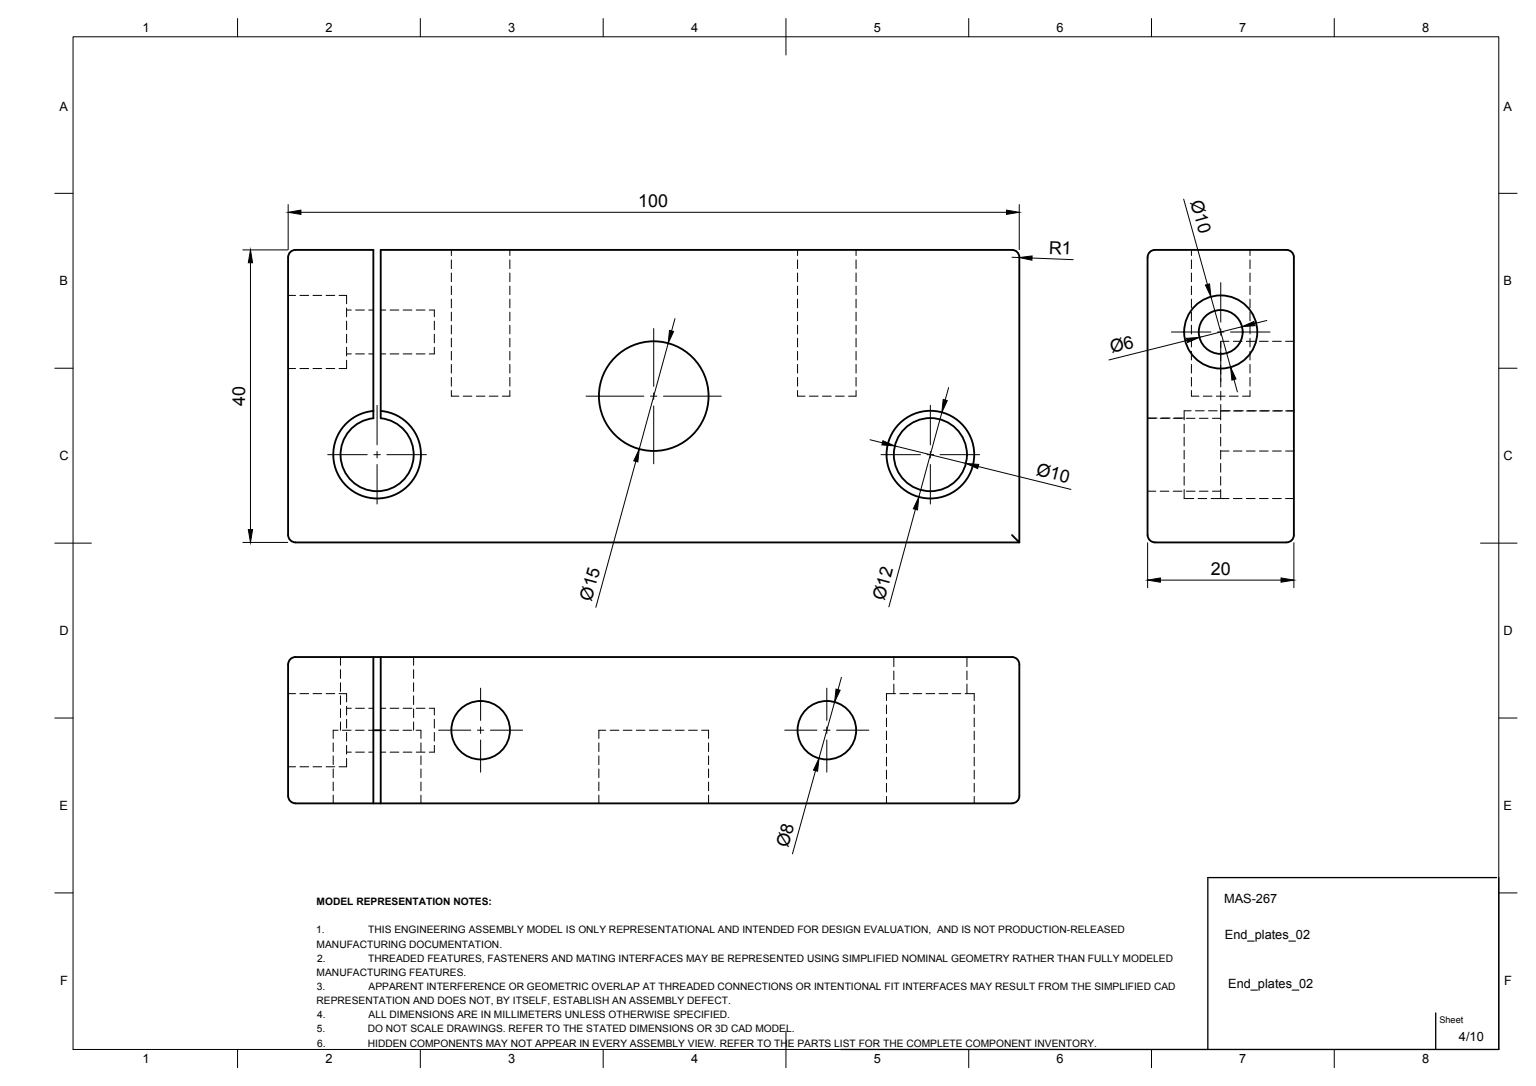
ISO-10303-21;
HEADER;
/* Generated by software containing ST-Developer
 * from STEP Tools, Inc. (www.steptools.com) 
 */

FILE_DESCRIPTION(
/* description */ (''),
/* implementation_level */ '2;1');

FILE_NAME(
/* name */ 'End_plates_02.step',
/* time_stamp */ '2026-10-12T15:29:24-07:00',
/* author */ (''),
/* organization */ (''),
/* preprocessor_version */ 'ST-DEVELOPER v20.2',
/* originating_system */ 'Autodesk Translation Framework v15.15.0.0',
/* authorisation */ '');

FILE_SCHEMA (('AUTOMOTIVE_DESIGN { 1 0 10303 214 3 1 1 }'));
ENDSEC;

DATA;
#10=MECHANICAL_DESIGN_GEOMETRIC_PRESENTATION_REPRESENTATION('',(#163),#9496);
#145=SHAPE_REPRESENTATION_RELATIONSHIP('SRR','None',#9539,#154);
#154=ADVANCED_BREP_SHAPE_REPRESENTATION('',(#220),#9487);
#163=STYLED_ITEM('',(#9593),#220);
#220=MANIFOLD_SOLID_BREP('Body1',#4965);
#277=ELLIPSE('',#5185,1.4142135623731,1.);
#278=ELLIPSE('',#5196,1.4142135623731,1.);
#279=SPHERICAL_SURFACE('',#5169,0.999999999999996);
#280=SPHERICAL_SURFACE('',#5173,0.999999999999996);
#281=SPHERICAL_SURFACE('',#5177,0.999999999999996);
#282=SPHERICAL_SURFACE('',#5181,0.999999999999996);
#283=SPHERICAL_SURFACE('',#5186,0.999999999999996);
#284=SPHERICAL_SURFACE('',#5192,0.999999999999996);
#333=FACE_BOUND('',#956,.T.);
#334=FACE_BOUND('',#963,.T.);
#335=FACE_BOUND('',#970,.T.);
#336=FACE_BOUND('',#972,.T.);
#337=FACE_BOUND('',#975,.T.);
#338=FACE_BOUND('',#978,.T.);
#339=FACE_BOUND('',#979,.T.);
#340=FACE_BOUND('',#1000,.T.);
#341=FACE_BOUND('',#1001,.T.);
#342=FACE_BOUND('',#1003,.T.);
#482=PLANE('',#5127);
#483=PLANE('',#5132);
#484=PLANE('',#5136);
#485=PLANE('',#5140);
#486=PLANE('',#5147);
#487=PLANE('',#5153);
#488=PLANE('',#5154);
#489=PLANE('',#5157);
#490=PLANE('',#5159);
#491=PLANE('',#5164);
#492=PLANE('',#5202);
#493=PLANE('',#5203);
#494=PLANE('',#5206);
#495=PLANE('',#5207);
#496=PLANE('',#5209);
#497=PLANE('',#5212);
#622=FACE_OUTER_BOUND('',#954,.T.);
#623=FACE_OUTER_BOUND('',#955,.T.);
#624=FACE_OUTER_BOUND('',#957,.T.);
#625=FACE_OUTER_BOUND('',#958,.T.);
#626=FACE_OUTER_BOUND('',#959,.T.);
#627=FACE_OUTER_BOUND('',#960,.T.);
#628=FACE_OUTER_BOUND('',#961,.T.);
#629=FACE_OUTER_BOUND('',#962,.T.);
#630=FACE_OUTER_BOUND('',#964,.T.);
#631=FACE_OUTER_BOUND('',#965,.T.);
#632=FACE_OUTER_BOUND('',#966,.T.);
#633=FACE_OUTER_BOUND('',#967,.T.);
#634=FACE_OUTER_BOUND('',#968,.T.);
#635=FACE_OUTER_BOUND('',#969,.T.);
#636=FACE_OUTER_BOUND('',#971,.T.);
#637=FACE_OUTER_BOUND('',#973,.T.);
#638=FACE_OUTER_BOUND('',#974,.T.);
#639=FACE_OUTER_BOUND('',#976,.T.);
#640=FACE_OUTER_BOUND('',#977,.T.);
#641=FACE_OUTER_BOUND('',#980,.T.);
#642=FACE_OUTER_BOUND('',#981,.T.);
#643=FACE_OUTER_BOUND('',#982,.T.);
#644=FACE_OUTER_BOUND('',#983,.T.);
#645=FACE_OUTER_BOUND('',#984,.T.);
#646=FACE_OUTER_BOUND('',#985,.T.);
#647=FACE_OUTER_BOUND('',#986,.T.);
#648=FACE_OUTER_BOUND('',#987,.T.);
#649=FACE_OUTER_BOUND('',#988,.T.);
#650=FACE_OUTER_BOUND('',#989,.T.);
#651=FACE_OUTER_BOUND('',#990,.T.);
#652=FACE_OUTER_BOUND('',#991,.T.);
#653=FACE_OUTER_BOUND('',#992,.T.);
#654=FACE_OUTER_BOUND('',#993,.T.);
#655=FACE_OUTER_BOUND('',#994,.T.);
#656=FACE_OUTER_BOUND('',#995,.T.);
#657=FACE_OUTER_BOUND('',#996,.T.);
#658=FACE_OUTER_BOUND('',#997,.T.);
#659=FACE_OUTER_BOUND('',#998,.T.);
#660=FACE_OUTER_BOUND('',#999,.T.);
#661=FACE_OUTER_BOUND('',#1002,.T.);
#662=FACE_OUTER_BOUND('',#1004,.T.);
#663=FACE_OUTER_BOUND('',#1005,.T.);
#664=FACE_OUTER_BOUND('',#1006,.T.);
#665=FACE_OUTER_BOUND('',#1007,.T.);
#666=FACE_OUTER_BOUND('',#1008,.T.);
#954=EDGE_LOOP('',(#3325,#3326,#3327,#3328));
#955=EDGE_LOOP('',(#3329));
#956=EDGE_LOOP('',(#3330));
#957=EDGE_LOOP('',(#3331,#3332,#3333,#3334));
#958=EDGE_LOOP('',(#3335));
#959=EDGE_LOOP('',(#3336,#3337,#3338,#3339));
#960=EDGE_LOOP('',(#3340));
#961=EDGE_LOOP('',(#3341,#3342,#3343,#3344));
#962=EDGE_LOOP('',(#3345));
#963=EDGE_LOOP('',(#3346));
#964=EDGE_LOOP('',(#3347,#3348,#3349,#3350));
#965=EDGE_LOOP('',(#3351,#3352,#3353,#3354));
#966=EDGE_LOOP('',(#3355));
#967=EDGE_LOOP('',(#3356,#3357,#3358,#3359));
#968=EDGE_LOOP('',(#3360,#3361,#3362,#3363));
#969=EDGE_LOOP('',(#3364,#3365,#3366,#3367,#3368,#3369,#3370,#3371));
#970=EDGE_LOOP('',(#3372));
#971=EDGE_LOOP('',(#3373,#3374,#3375,#3376,#3377,#3378,#3379,#3380));
#972=EDGE_LOOP('',(#3381));
#973=EDGE_LOOP('',(#3382,#3383,#3384,#3385));
#974=EDGE_LOOP('',(#3386,#3387,#3388,#3389,#3390,#3391,#3392,#3393));
#975=EDGE_LOOP('',(#3394));
#976=EDGE_LOOP('',(#3395,#3396,#3397,#3398));
#977=EDGE_LOOP('',(#3399,#3400,#3401,#3402));
#978=EDGE_LOOP('',(#3403));
#979=EDGE_LOOP('',(#3404));
#980=EDGE_LOOP('',(#3405,#3406,#3407,#3408));
#981=EDGE_LOOP('',(#3409,#3410,#3411,#3412));
#982=EDGE_LOOP('',(#3413,#3414,#3415));
#983=EDGE_LOOP('',(#3416,#3417,#3418));
#984=EDGE_LOOP('',(#3419,#3420,#3421,#3422));
#985=EDGE_LOOP('',(#3423,#3424,#3425));
#986=EDGE_LOOP('',(#3426,#3427,#3428));
#987=EDGE_LOOP('',(#3429,#3430,#3431,#3432));
#988=EDGE_LOOP('',(#3433,#3434,#3435));
#989=EDGE_LOOP('',(#3436,#3437,#3438,#3439));
#990=EDGE_LOOP('',(#3440,#3441,#3442,#3443));
#991=EDGE_LOOP('',(#3444,#3445,#3446));
#992=EDGE_LOOP('',(#3447,#3448,#3449,#3450));
#993=EDGE_LOOP('',(#3451,#3452,#3453,#3454));
#994=EDGE_LOOP('',(#3455,#3456,#3457,#3458));
#995=EDGE_LOOP('',(#3459,#3460,#3461,#3462));
#996=EDGE_LOOP('',(#3463,#3464,#3465,#3466));
#997=EDGE_LOOP('',(#3467,#3468,#3469,#3470));
#998=EDGE_LOOP('',(#3471,#3472,#3473,#3474));
#999=EDGE_LOOP('',(#3475,#3476,#3477,#3478,#3479,#3480,#3481,#3482));
#1000=EDGE_LOOP('',(#3483));
#1001=EDGE_LOOP('',(#3484));
#1002=EDGE_LOOP('',(#3485,#3486,#3487,#3488));
#1003=EDGE_LOOP('',(#3489));
#1004=EDGE_LOOP('',(#3490,#3491,#3492,#3493));
#1005=EDGE_LOOP('',(#3494,#3495,#3496,#3497));
#1006=EDGE_LOOP('',(#3498));
#1007=EDGE_LOOP('',(#3499,#3500,#3501,#3502));
#1008=EDGE_LOOP('',(#3503,#3504,#3505,#3506));
#1435=LINE('',#7477,#1672);
#1436=LINE('',#7486,#1673);
#1437=LINE('',#7493,#1674);
#1438=LINE('',#7500,#1675);
#1439=LINE('',#7507,#1676);
#1440=LINE('',#7513,#1677);
#1441=LINE('',#7518,#1678);
#1442=LINE('',#7523,#1679);
#1443=LINE('',#7527,#1680);
#1444=LINE('',#7531,#1681);
#1445=LINE('',#7533,#1682);
#1446=LINE('',#7535,#1683);
#1447=LINE('',#7537,#1684);
#1448=LINE('',#7539,#1685);
#1449=LINE('',#7541,#1686);
#1450=LINE('',#7542,#1687);
#1451=LINE('',#7545,#1688);
#1452=LINE('',#7547,#1689);
#1453=LINE('',#7549,#1690);
#1454=LINE('',#7553,#1691);
#1455=LINE('',#7557,#1692);
#1456=LINE('',#7563,#1693);
#1457=LINE('',#7567,#1694);
#1458=LINE('',#7568,#1695);
#1459=LINE('',#7571,#1696);
#1460=LINE('',#7575,#1697);
#1461=LINE('',#7576,#1698);
#1462=LINE('',#7579,#1699);
#1463=LINE('',#7583,#1700);
#1464=LINE('',#7586,#1701);
#1465=LINE('',#7599,#1702);
#1466=LINE('',#7600,#1703);
#1467=LINE('',#7613,#1704);
#1468=LINE('',#7615,#1705);
#1469=LINE('',#7624,#1706);
#1470=LINE('',#7626,#1707);
#1471=LINE('',#7627,#1708);
#1472=LINE('',#7634,#1709);
#1473=LINE('',#7637,#1710);
#1474=LINE('',#7639,#1711);
#1475=LINE('',#7641,#1712);
#1476=LINE('',#7643,#1713);
#1477=LINE('',#7644,#1714);
#1478=LINE('',#7646,#1715);
#1479=LINE('',#7647,#1716);
#1480=LINE('',#7649,#1717);
#1481=LINE('',#7661,#1718);
#1672=VECTOR('',#5834,6.00000000000001);
#1673=VECTOR('',#5845,4.);
#1674=VECTOR('',#5854,4.);
#1675=VECTOR('',#5863,5.);
#1676=VECTOR('',#5872,3.00000000000001);
#1677=VECTOR('',#5879,3.00000000000001);
#1678=VECTOR('',#5886,4.99999999999977);
#1679=VECTOR('',#5891,10.);
#1680=VECTOR('',#5894,10.);
#1681=VECTOR('',#5899,10.);
#1682=VECTOR('',#5900,10.);
#1683=VECTOR('',#5901,10.);
#1684=VECTOR('',#5902,10.);
#1685=VECTOR('',#5903,10.);
#1686=VECTOR('',#5904,10.);
#1687=VECTOR('',#5905,10.);
#1688=VECTOR('',#5908,10.);
#1689=VECTOR('',#5909,10.);
#1690=VECTOR('',#5910,10.);
#1691=VECTOR('',#5913,10.);
#1692=VECTOR('',#5918,10.);
#1693=VECTOR('',#5925,10.);
#1694=VECTOR('',#5928,10.);
#1695=VECTOR('',#5929,10.);
#1696=VECTOR('',#5932,10.);
#1697=VECTOR('',#5937,10.);
#1698=VECTOR('',#5938,10.);
#1699=VECTOR('',#5941,10.);
#1700=VECTOR('',#5946,10.);
#1701=VECTOR('',#5949,10.);
#1702=VECTOR('',#5966,10.);
#1703=VECTOR('',#5967,10.);
#1704=VECTOR('',#5984,10.);
#1705=VECTOR('',#5985,10.);
#1706=VECTOR('',#5998,10.);
#1707=VECTOR('',#6001,10.);
#1708=VECTOR('',#6002,10.);
#1709=VECTOR('',#6011,10.);
#1710=VECTOR('',#6016,10.);
#1711=VECTOR('',#6019,10.);
#1712=VECTOR('',#6022,10.);
#1713=VECTOR('',#6025,10.);
#1714=VECTOR('',#6026,10.);
#1715=VECTOR('',#6029,10.);
#1716=VECTOR('',#6030,10.);
#1717=VECTOR('',#6033,10.);
#1718=VECTOR('',#6052,7.50000000000001);
#1909=CIRCLE('',#5125,6.00000000000001);
#1910=CIRCLE('',#5126,6.00000000000001);
#1911=CIRCLE('',#5128,4.99999999999977);
#1912=CIRCLE('',#5130,4.);
#1913=CIRCLE('',#5131,4.);
#1914=CIRCLE('',#5134,4.);
#1915=CIRCLE('',#5135,4.);
#1916=CIRCLE('',#5138,5.);
#1917=CIRCLE('',#5139,5.);
#1918=CIRCLE('',#5141,3.00000000000001);
#1919=CIRCLE('',#5143,3.00000000000001);
#1920=CIRCLE('',#5145,3.00000000000001);
#1921=CIRCLE('',#5146,3.00000000000001);
#1922=CIRCLE('',#5149,4.99999999999977);
#1923=CIRCLE('',#5151,4.99999999999977);
#1924=CIRCLE('',#5152,4.99999999999977);
#1925=CIRCLE('',#5155,1.);
#1926=CIRCLE('',#5156,1.);
#1927=CIRCLE('',#5158,6.00000000000001);
#1928=CIRCLE('',#5160,1.);
#1929=CIRCLE('',#5161,1.);
#1930=CIRCLE('',#5163,1.);
#1931=CIRCLE('',#5166,0.999999999999996);
#1932=CIRCLE('',#5168,1.);
#1933=CIRCLE('',#5170,0.999999999999996);
#1934=CIRCLE('',#5171,0.999999999999996);
#1935=CIRCLE('',#5172,1.);
#1936=CIRCLE('',#5174,0.999999999999996);
#1937=CIRCLE('',#5175,0.999999999999996);
#1938=CIRCLE('',#5178,0.999999999999996);
#1939=CIRCLE('',#5179,0.999999999999996);
#1940=CIRCLE('',#5180,1.);
#1941=CIRCLE('',#5182,0.999999999999996);
#1942=CIRCLE('',#5183,1.);
#1943=CIRCLE('',#5187,0.999999999999996);
#1944=CIRCLE('',#5188,0.999999999999996);
#1945=CIRCLE('',#5189,1.);
#1946=CIRCLE('',#5193,0.999999999999996);
#1947=CIRCLE('',#5194,0.999999999999996);
#1948=CIRCLE('',#5204,6.00000000000001);
#1949=CIRCLE('',#5205,7.50000000000001);
#1950=CIRCLE('',#5210,7.50000000000001);
#2264=VERTEX_POINT('',#7474);
#2265=VERTEX_POINT('',#7476);
#2266=VERTEX_POINT('',#7480);
#2267=VERTEX_POINT('',#7483);
#2268=VERTEX_POINT('',#7485);
#2269=VERTEX_POINT('',#7490);
#2270=VERTEX_POINT('',#7492);
#2271=VERTEX_POINT('',#7497);
#2272=VERTEX_POINT('',#7499);
#2273=VERTEX_POINT('',#7503);
#2274=VERTEX_POINT('',#7506);
#2275=VERTEX_POINT('',#7510);
#2276=VERTEX_POINT('',#7512);
#2277=VERTEX_POINT('',#7517);
#2278=VERTEX_POINT('',#7521);
#2279=VERTEX_POINT('',#7522);
#2280=VERTEX_POINT('',#7524);
#2281=VERTEX_POINT('',#7526);
#2282=VERTEX_POINT('',#7530);
#2283=VERTEX_POINT('',#7532);
#2284=VERTEX_POINT('',#7534);
#2285=VERTEX_POINT('',#7536);
#2286=VERTEX_POINT('',#7538);
#2287=VERTEX_POINT('',#7540);
#2288=VERTEX_POINT('',#7544);
#2289=VERTEX_POINT('',#7546);
#2290=VERTEX_POINT('',#7548);
#2291=VERTEX_POINT('',#7550);
#2292=VERTEX_POINT('',#7552);
#2293=VERTEX_POINT('',#7556);
#2294=VERTEX_POINT('',#7560);
#2295=VERTEX_POINT('',#7562);
#2296=VERTEX_POINT('',#7564);
#2297=VERTEX_POINT('',#7566);
#2298=VERTEX_POINT('',#7570);
#2299=VERTEX_POINT('',#7574);
#2300=VERTEX_POINT('',#7578);
#2301=VERTEX_POINT('',#7582);
#2302=VERTEX_POINT('',#7584);
#2303=VERTEX_POINT('',#7588);
#2304=VERTEX_POINT('',#7589);
#2305=VERTEX_POINT('',#7591);
#2306=VERTEX_POINT('',#7595);
#2307=VERTEX_POINT('',#7602);
#2308=VERTEX_POINT('',#7603);
#2309=VERTEX_POINT('',#7608);
#2310=VERTEX_POINT('',#7612);
#2311=VERTEX_POINT('',#7614);
#2312=VERTEX_POINT('',#7618);
#2313=VERTEX_POINT('',#7620);
#2314=VERTEX_POINT('',#7629);
#2315=VERTEX_POINT('',#7633);
#2316=VERTEX_POINT('',#7652);
#2317=VERTEX_POINT('',#7658);
#2715=EDGE_CURVE('',#2264,#2264,#1909,.T.);
#2716=EDGE_CURVE('',#2264,#2265,#1435,.T.);
#2717=EDGE_CURVE('',#2265,#2265,#1910,.T.);
#2718=EDGE_CURVE('',#2266,#2266,#1911,.T.);
#2719=EDGE_CURVE('',#2267,#2267,#1912,.T.);
#2720=EDGE_CURVE('',#2267,#2268,#1436,.T.);
#2721=EDGE_CURVE('',#2268,#2268,#1913,.T.);
#2722=EDGE_CURVE('',#2269,#2269,#1914,.T.);
#2723=EDGE_CURVE('',#2269,#2270,#1437,.T.);
#2724=EDGE_CURVE('',#2270,#2270,#1915,.T.);
#2725=EDGE_CURVE('',#2271,#2271,#1916,.T.);
#2726=EDGE_CURVE('',#2271,#2272,#1438,.T.);
#2727=EDGE_CURVE('',#2272,#2272,#1917,.T.);
#2728=EDGE_CURVE('',#2273,#2273,#1918,.T.);
#2729=EDGE_CURVE('',#2273,#2274,#1439,.T.);
#2730=EDGE_CURVE('',#2274,#2274,#1919,.T.);
#2731=EDGE_CURVE('',#2275,#2275,#1920,.T.);
#2732=EDGE_CURVE('',#2275,#2276,#1440,.T.);
#2733=EDGE_CURVE('',#2276,#2276,#1921,.T.);
#2734=EDGE_CURVE('',#2266,#2277,#1441,.T.);
#2735=EDGE_CURVE('',#2277,#2277,#1922,.T.);
#2736=EDGE_CURVE('',#2278,#2279,#1442,.T.);
#2737=EDGE_CURVE('',#2280,#2278,#1923,.T.);
#2738=EDGE_CURVE('',#2281,#2280,#1443,.T.);
#2739=EDGE_CURVE('',#2279,#2281,#1924,.T.);
#2740=EDGE_CURVE('',#2281,#2282,#1444,.T.);
#2741=EDGE_CURVE('',#2283,#2282,#1445,.T.);
#2742=EDGE_CURVE('',#2284,#2283,#1446,.T.);
#2743=EDGE_CURVE('',#2285,#2284,#1447,.T.);
#2744=EDGE_CURVE('',#2286,#2285,#1448,.T.);
#2745=EDGE_CURVE('',#2287,#2286,#1449,.T.);
#2746=EDGE_CURVE('',#2287,#2279,#1450,.T.);
#2747=EDGE_CURVE('',#2288,#2280,#1451,.T.);
#2748=EDGE_CURVE('',#2289,#2288,#1452,.T.);
#2749=EDGE_CURVE('',#2290,#2289,#1453,.T.);
#2750=EDGE_CURVE('',#2291,#2290,#1925,.T.);
#2751=EDGE_CURVE('',#2292,#2291,#1454,.T.);
#2752=EDGE_CURVE('',#2282,#2292,#1926,.T.);
#2753=EDGE_CURVE('',#2278,#2293,#1455,.T.);
#2754=EDGE_CURVE('',#2288,#2293,#1927,.T.);
#2755=EDGE_CURVE('',#2294,#2287,#1928,.T.);
#2756=EDGE_CURVE('',#2295,#2294,#1456,.T.);
#2757=EDGE_CURVE('',#2296,#2295,#1929,.T.);
#2758=EDGE_CURVE('',#2297,#2296,#1457,.T.);
#2759=EDGE_CURVE('',#2293,#2297,#1458,.T.);
#2760=EDGE_CURVE('',#2292,#2298,#1459,.T.);
#2761=EDGE_CURVE('',#2298,#2283,#1930,.F.);
#2762=EDGE_CURVE('',#2299,#2291,#1460,.T.);
#2763=EDGE_CURVE('',#2298,#2299,#1461,.T.);
#2764=EDGE_CURVE('',#2290,#2300,#1462,.T.);
#2765=EDGE_CURVE('',#2300,#2299,#1931,.F.);
#2766=EDGE_CURVE('',#2295,#2301,#1463,.T.);
#2767=EDGE_CURVE('',#2301,#2302,#1932,.F.);
#2768=EDGE_CURVE('',#2302,#2296,#1464,.T.);
#2769=EDGE_CURVE('',#2303,#2304,#1933,.F.);
#2770=EDGE_CURVE('',#2305,#2303,#1934,.F.);
#2771=EDGE_CURVE('',#2304,#2305,#1935,.F.);
#2772=EDGE_CURVE('',#2306,#2301,#1936,.F.);
#2773=EDGE_CURVE('',#2302,#2306,#1937,.F.);
#2774=EDGE_CURVE('',#2306,#2305,#1465,.T.);
#2775=EDGE_CURVE('',#2303,#2302,#1466,.T.);
#2776=EDGE_CURVE('',#2307,#2308,#1938,.F.);
#2777=EDGE_CURVE('',#2285,#2307,#1939,.F.);
#2778=EDGE_CURVE('',#2308,#2285,#1940,.F.);
#2779=EDGE_CURVE('',#2309,#2300,#1941,.F.);
#2780=EDGE_CURVE('',#2299,#2309,#1942,.F.);
#2781=EDGE_CURVE('',#2310,#2309,#1467,.T.);
#2782=EDGE_CURVE('',#2300,#2311,#1468,.T.);
#2783=EDGE_CURVE('',#2311,#2310,#277,.T.);
#2784=EDGE_CURVE('',#2286,#2312,#1943,.F.);
#2785=EDGE_CURVE('',#2313,#2286,#1944,.F.);
#2786=EDGE_CURVE('',#2312,#2313,#1945,.F.);
#2787=EDGE_CURVE('',#2307,#2313,#1469,.T.);
#2788=EDGE_CURVE('',#2301,#2312,#1470,.T.);
#2789=EDGE_CURVE('',#2313,#2306,#1471,.T.);
#2790=EDGE_CURVE('',#2314,#2298,#1946,.F.);
#2791=EDGE_CURVE('',#2283,#2314,#1947,.F.);
#2792=EDGE_CURVE('',#2314,#2315,#1472,.T.);
#2793=EDGE_CURVE('',#2315,#2284,#278,.T.);
#2794=EDGE_CURVE('',#2312,#2294,#1473,.T.);
#2795=EDGE_CURVE('',#2309,#2314,#1474,.T.);
#2796=EDGE_CURVE('',#2315,#2308,#1475,.T.);
#2797=EDGE_CURVE('',#2308,#2304,#1476,.T.);
#2798=EDGE_CURVE('',#2305,#2307,#1477,.T.);
#2799=EDGE_CURVE('',#2311,#2303,#1478,.T.);
#2800=EDGE_CURVE('',#2304,#2310,#1479,.T.);
#2801=EDGE_CURVE('',#2315,#2310,#1480,.T.);
#2802=EDGE_CURVE('',#2289,#2297,#1948,.T.);
#2803=EDGE_CURVE('',#2316,#2316,#1949,.T.);
#2804=EDGE_CURVE('',#2317,#2317,#1950,.T.);
#2805=EDGE_CURVE('',#2317,#2316,#1481,.T.);
#3325=ORIENTED_EDGE('',*,*,#2715,.F.);
#3326=ORIENTED_EDGE('',*,*,#2716,.T.);
#3327=ORIENTED_EDGE('',*,*,#2717,.T.);
#3328=ORIENTED_EDGE('',*,*,#2716,.F.);
#3329=ORIENTED_EDGE('',*,*,#2717,.F.);
#3330=ORIENTED_EDGE('',*,*,#2718,.F.);
#3331=ORIENTED_EDGE('',*,*,#2719,.F.);
#3332=ORIENTED_EDGE('',*,*,#2720,.T.);
#3333=ORIENTED_EDGE('',*,*,#2721,.T.);
#3334=ORIENTED_EDGE('',*,*,#2720,.F.);
#3335=ORIENTED_EDGE('',*,*,#2721,.F.);
#3336=ORIENTED_EDGE('',*,*,#2722,.F.);
#3337=ORIENTED_EDGE('',*,*,#2723,.T.);
#3338=ORIENTED_EDGE('',*,*,#2724,.T.);
#3339=ORIENTED_EDGE('',*,*,#2723,.F.);
#3340=ORIENTED_EDGE('',*,*,#2724,.F.);
#3341=ORIENTED_EDGE('',*,*,#2725,.F.);
#3342=ORIENTED_EDGE('',*,*,#2726,.T.);
#3343=ORIENTED_EDGE('',*,*,#2727,.T.);
#3344=ORIENTED_EDGE('',*,*,#2726,.F.);
#3345=ORIENTED_EDGE('',*,*,#2727,.F.);
#3346=ORIENTED_EDGE('',*,*,#2728,.F.);
#3347=ORIENTED_EDGE('',*,*,#2728,.T.);
#3348=ORIENTED_EDGE('',*,*,#2729,.T.);
#3349=ORIENTED_EDGE('',*,*,#2730,.F.);
#3350=ORIENTED_EDGE('',*,*,#2729,.F.);
#3351=ORIENTED_EDGE('',*,*,#2731,.F.);
#3352=ORIENTED_EDGE('',*,*,#2732,.T.);
#3353=ORIENTED_EDGE('',*,*,#2733,.T.);
#3354=ORIENTED_EDGE('',*,*,#2732,.F.);
#3355=ORIENTED_EDGE('',*,*,#2733,.F.);
#3356=ORIENTED_EDGE('',*,*,#2718,.T.);
#3357=ORIENTED_EDGE('',*,*,#2734,.T.);
#3358=ORIENTED_EDGE('',*,*,#2735,.F.);
#3359=ORIENTED_EDGE('',*,*,#2734,.F.);
#3360=ORIENTED_EDGE('',*,*,#2736,.F.);
#3361=ORIENTED_EDGE('',*,*,#2737,.F.);
#3362=ORIENTED_EDGE('',*,*,#2738,.F.);
#3363=ORIENTED_EDGE('',*,*,#2739,.F.);
#3364=ORIENTED_EDGE('',*,*,#2739,.T.);
#3365=ORIENTED_EDGE('',*,*,#2740,.T.);
#3366=ORIENTED_EDGE('',*,*,#2741,.F.);
#3367=ORIENTED_EDGE('',*,*,#2742,.F.);
#3368=ORIENTED_EDGE('',*,*,#2743,.F.);
#3369=ORIENTED_EDGE('',*,*,#2744,.F.);
#3370=ORIENTED_EDGE('',*,*,#2745,.F.);
#3371=ORIENTED_EDGE('',*,*,#2746,.T.);
#3372=ORIENTED_EDGE('',*,*,#2735,.T.);
#3373=ORIENTED_EDGE('',*,*,#2738,.T.);
#3374=ORIENTED_EDGE('',*,*,#2747,.F.);
#3375=ORIENTED_EDGE('',*,*,#2748,.F.);
#3376=ORIENTED_EDGE('',*,*,#2749,.F.);
#3377=ORIENTED_EDGE('',*,*,#2750,.F.);
#3378=ORIENTED_EDGE('',*,*,#2751,.F.);
#3379=ORIENTED_EDGE('',*,*,#2752,.F.);
#3380=ORIENTED_EDGE('',*,*,#2740,.F.);
#3381=ORIENTED_EDGE('',*,*,#2731,.T.);
#3382=ORIENTED_EDGE('',*,*,#2737,.T.);
#3383=ORIENTED_EDGE('',*,*,#2753,.T.);
#3384=ORIENTED_EDGE('',*,*,#2754,.F.);
#3385=ORIENTED_EDGE('',*,*,#2747,.T.);
#3386=ORIENTED_EDGE('',*,*,#2736,.T.);
#3387=ORIENTED_EDGE('',*,*,#2746,.F.);
#3388=ORIENTED_EDGE('',*,*,#2755,.F.);
#3389=ORIENTED_EDGE('',*,*,#2756,.F.);
#3390=ORIENTED_EDGE('',*,*,#2757,.F.);
#3391=ORIENTED_EDGE('',*,*,#2758,.F.);
#3392=ORIENTED_EDGE('',*,*,#2759,.F.);
#3393=ORIENTED_EDGE('',*,*,#2753,.F.);
#3394=ORIENTED_EDGE('',*,*,#2730,.T.);
#3395=ORIENTED_EDGE('',*,*,#2752,.T.);
#3396=ORIENTED_EDGE('',*,*,#2760,.T.);
#3397=ORIENTED_EDGE('',*,*,#2761,.T.);
#3398=ORIENTED_EDGE('',*,*,#2741,.T.);
#3399=ORIENTED_EDGE('',*,*,#2751,.T.);
#3400=ORIENTED_EDGE('',*,*,#2762,.F.);
#3401=ORIENTED_EDGE('',*,*,#2763,.F.);
#3402=ORIENTED_EDGE('',*,*,#2760,.F.);
#3403=ORIENTED_EDGE('',*,*,#2719,.T.);
#3404=ORIENTED_EDGE('',*,*,#2722,.T.);
#3405=ORIENTED_EDGE('',*,*,#2750,.T.);
#3406=ORIENTED_EDGE('',*,*,#2764,.T.);
#3407=ORIENTED_EDGE('',*,*,#2765,.T.);
#3408=ORIENTED_EDGE('',*,*,#2762,.T.);
#3409=ORIENTED_EDGE('',*,*,#2757,.T.);
#3410=ORIENTED_EDGE('',*,*,#2766,.T.);
#3411=ORIENTED_EDGE('',*,*,#2767,.T.);
#3412=ORIENTED_EDGE('',*,*,#2768,.T.);
#3413=ORIENTED_EDGE('',*,*,#2769,.F.);
#3414=ORIENTED_EDGE('',*,*,#2770,.F.);
#3415=ORIENTED_EDGE('',*,*,#2771,.F.);
#3416=ORIENTED_EDGE('',*,*,#2772,.F.);
#3417=ORIENTED_EDGE('',*,*,#2773,.F.);
#3418=ORIENTED_EDGE('',*,*,#2767,.F.);
#3419=ORIENTED_EDGE('',*,*,#2773,.T.);
#3420=ORIENTED_EDGE('',*,*,#2774,.T.);
#3421=ORIENTED_EDGE('',*,*,#2770,.T.);
#3422=ORIENTED_EDGE('',*,*,#2775,.T.);
#3423=ORIENTED_EDGE('',*,*,#2776,.F.);
#3424=ORIENTED_EDGE('',*,*,#2777,.F.);
#3425=ORIENTED_EDGE('',*,*,#2778,.F.);
#3426=ORIENTED_EDGE('',*,*,#2765,.F.);
#3427=ORIENTED_EDGE('',*,*,#2779,.F.);
#3428=ORIENTED_EDGE('',*,*,#2780,.F.);
#3429=ORIENTED_EDGE('',*,*,#2781,.T.);
#3430=ORIENTED_EDGE('',*,*,#2779,.T.);
#3431=ORIENTED_EDGE('',*,*,#2782,.T.);
#3432=ORIENTED_EDGE('',*,*,#2783,.T.);
#3433=ORIENTED_EDGE('',*,*,#2784,.F.);
#3434=ORIENTED_EDGE('',*,*,#2785,.F.);
#3435=ORIENTED_EDGE('',*,*,#2786,.F.);
#3436=ORIENTED_EDGE('',*,*,#2777,.T.);
#3437=ORIENTED_EDGE('',*,*,#2787,.T.);
#3438=ORIENTED_EDGE('',*,*,#2785,.T.);
#3439=ORIENTED_EDGE('',*,*,#2744,.T.);
#3440=ORIENTED_EDGE('',*,*,#2772,.T.);
#3441=ORIENTED_EDGE('',*,*,#2788,.T.);
#3442=ORIENTED_EDGE('',*,*,#2786,.T.);
#3443=ORIENTED_EDGE('',*,*,#2789,.T.);
#3444=ORIENTED_EDGE('',*,*,#2790,.F.);
#3445=ORIENTED_EDGE('',*,*,#2791,.F.);
#3446=ORIENTED_EDGE('',*,*,#2761,.F.);
#3447=ORIENTED_EDGE('',*,*,#2742,.T.);
#3448=ORIENTED_EDGE('',*,*,#2791,.T.);
#3449=ORIENTED_EDGE('',*,*,#2792,.T.);
#3450=ORIENTED_EDGE('',*,*,#2793,.T.);
#3451=ORIENTED_EDGE('',*,*,#2755,.T.);
#3452=ORIENTED_EDGE('',*,*,#2745,.T.);
#3453=ORIENTED_EDGE('',*,*,#2784,.T.);
#3454=ORIENTED_EDGE('',*,*,#2794,.T.);
#3455=ORIENTED_EDGE('',*,*,#2790,.T.);
#3456=ORIENTED_EDGE('',*,*,#2763,.T.);
#3457=ORIENTED_EDGE('',*,*,#2780,.T.);
#3458=ORIENTED_EDGE('',*,*,#2795,.T.);
#3459=ORIENTED_EDGE('',*,*,#2796,.T.);
#3460=ORIENTED_EDGE('',*,*,#2778,.T.);
#3461=ORIENTED_EDGE('',*,*,#2743,.T.);
#3462=ORIENTED_EDGE('',*,*,#2793,.F.);
#3463=ORIENTED_EDGE('',*,*,#2776,.T.);
#3464=ORIENTED_EDGE('',*,*,#2797,.T.);
#3465=ORIENTED_EDGE('',*,*,#2771,.T.);
#3466=ORIENTED_EDGE('',*,*,#2798,.T.);
#3467=ORIENTED_EDGE('',*,*,#2799,.T.);
#3468=ORIENTED_EDGE('',*,*,#2769,.T.);
#3469=ORIENTED_EDGE('',*,*,#2800,.T.);
#3470=ORIENTED_EDGE('',*,*,#2783,.F.);
#3471=ORIENTED_EDGE('',*,*,#2800,.F.);
#3472=ORIENTED_EDGE('',*,*,#2797,.F.);
#3473=ORIENTED_EDGE('',*,*,#2796,.F.);
#3474=ORIENTED_EDGE('',*,*,#2801,.T.);
#3475=ORIENTED_EDGE('',*,*,#2758,.T.);
#3476=ORIENTED_EDGE('',*,*,#2768,.F.);
#3477=ORIENTED_EDGE('',*,*,#2775,.F.);
#3478=ORIENTED_EDGE('',*,*,#2799,.F.);
#3479=ORIENTED_EDGE('',*,*,#2782,.F.);
#3480=ORIENTED_EDGE('',*,*,#2764,.F.);
#3481=ORIENTED_EDGE('',*,*,#2749,.T.);
#3482=ORIENTED_EDGE('',*,*,#2802,.T.);
#3483=ORIENTED_EDGE('',*,*,#2715,.T.);
#3484=ORIENTED_EDGE('',*,*,#2803,.T.);
#3485=ORIENTED_EDGE('',*,*,#2787,.F.);
#3486=ORIENTED_EDGE('',*,*,#2798,.F.);
#3487=ORIENTED_EDGE('',*,*,#2774,.F.);
#3488=ORIENTED_EDGE('',*,*,#2789,.F.);
#3489=ORIENTED_EDGE('',*,*,#2725,.T.);
#3490=ORIENTED_EDGE('',*,*,#2756,.T.);
#3491=ORIENTED_EDGE('',*,*,#2794,.F.);
#3492=ORIENTED_EDGE('',*,*,#2788,.F.);
#3493=ORIENTED_EDGE('',*,*,#2766,.F.);
#3494=ORIENTED_EDGE('',*,*,#2759,.T.);
#3495=ORIENTED_EDGE('',*,*,#2802,.F.);
#3496=ORIENTED_EDGE('',*,*,#2748,.T.);
#3497=ORIENTED_EDGE('',*,*,#2754,.T.);
#3498=ORIENTED_EDGE('',*,*,#2804,.F.);
#3499=ORIENTED_EDGE('',*,*,#2804,.T.);
#3500=ORIENTED_EDGE('',*,*,#2805,.T.);
#3501=ORIENTED_EDGE('',*,*,#2803,.F.);
#3502=ORIENTED_EDGE('',*,*,#2805,.F.);
#3503=ORIENTED_EDGE('',*,*,#2781,.F.);
#3504=ORIENTED_EDGE('',*,*,#2801,.F.);
#3505=ORIENTED_EDGE('',*,*,#2792,.F.);
#3506=ORIENTED_EDGE('',*,*,#2795,.F.);
#4545=CYLINDRICAL_SURFACE('',#5124,6.00000000000001);
#4546=CYLINDRICAL_SURFACE('',#5129,4.);
#4547=CYLINDRICAL_SURFACE('',#5133,4.);
#4548=CYLINDRICAL_SURFACE('',#5137,5.);
#4549=CYLINDRICAL_SURFACE('',#5142,3.00000000000001);
#4550=CYLINDRICAL_SURFACE('',#5144,3.00000000000001);
#4551=CYLINDRICAL_SURFACE('',#5148,4.99999999999977);
#4552=CYLINDRICAL_SURFACE('',#5150,4.99999999999977);
#4553=CYLINDRICAL_SURFACE('',#5162,1.);
#4554=CYLINDRICAL_SURFACE('',#5165,1.);
#4555=CYLINDRICAL_SURFACE('',#5167,1.);
#4556=CYLINDRICAL_SURFACE('',#5176,1.);
#4557=CYLINDRICAL_SURFACE('',#5184,1.);
#4558=CYLINDRICAL_SURFACE('',#5190,1.);
#4559=CYLINDRICAL_SURFACE('',#5191,1.);
#4560=CYLINDRICAL_SURFACE('',#5195,1.);
#4561=CYLINDRICAL_SURFACE('',#5197,1.);
#4562=CYLINDRICAL_SURFACE('',#5198,1.);
#4563=CYLINDRICAL_SURFACE('',#5199,1.);
#4564=CYLINDRICAL_SURFACE('',#5200,1.);
#4565=CYLINDRICAL_SURFACE('',#5201,1.);
#4566=CYLINDRICAL_SURFACE('',#5208,6.00000000000001);
#4567=CYLINDRICAL_SURFACE('',#5211,7.50000000000001);
#4633=ADVANCED_FACE('',(#622),#4545,.F.);
#4634=ADVANCED_FACE('',(#623,#333),#482,.T.);
#4635=ADVANCED_FACE('',(#624),#4546,.F.);
#4636=ADVANCED_FACE('',(#625),#483,.T.);
#4637=ADVANCED_FACE('',(#626),#4547,.F.);
#4638=ADVANCED_FACE('',(#627),#484,.T.);
#4639=ADVANCED_FACE('',(#628),#4548,.F.);
#4640=ADVANCED_FACE('',(#629,#334),#485,.T.);
#4641=ADVANCED_FACE('',(#630),#4549,.F.);
#4642=ADVANCED_FACE('',(#631),#4550,.F.);
#4643=ADVANCED_FACE('',(#632),#486,.T.);
#4644=ADVANCED_FACE('',(#633),#4551,.F.);
#4645=ADVANCED_FACE('',(#634),#4552,.F.);
#4646=ADVANCED_FACE('',(#635,#335),#487,.T.);
#4647=ADVANCED_FACE('',(#636,#336),#488,.F.);
#4648=ADVANCED_FACE('',(#637),#489,.T.);
#4649=ADVANCED_FACE('',(#638,#337),#490,.F.);
#4650=ADVANCED_FACE('',(#639),#4553,.T.);
#4651=ADVANCED_FACE('',(#640,#338,#339),#491,.T.);
#4652=ADVANCED_FACE('',(#641),#4554,.T.);
#4653=ADVANCED_FACE('',(#642),#4555,.T.);
#4654=ADVANCED_FACE('',(#643),#279,.T.);
#4655=ADVANCED_FACE('',(#644),#280,.T.);
#4656=ADVANCED_FACE('',(#645),#4556,.T.);
#4657=ADVANCED_FACE('',(#646),#281,.T.);
#4658=ADVANCED_FACE('',(#647),#282,.T.);
#4659=ADVANCED_FACE('',(#648),#4557,.T.);
#4660=ADVANCED_FACE('',(#649),#283,.T.);
#4661=ADVANCED_FACE('',(#650),#4558,.T.);
#4662=ADVANCED_FACE('',(#651),#4559,.T.);
#4663=ADVANCED_FACE('',(#652),#284,.T.);
#4664=ADVANCED_FACE('',(#653),#4560,.T.);
#4665=ADVANCED_FACE('',(#654),#4561,.T.);
#4666=ADVANCED_FACE('',(#655),#4562,.T.);
#4667=ADVANCED_FACE('',(#656),#4563,.T.);
#4668=ADVANCED_FACE('',(#657),#4564,.T.);
#4669=ADVANCED_FACE('',(#658),#4565,.T.);
#4670=ADVANCED_FACE('',(#659),#492,.T.);
#4671=ADVANCED_FACE('',(#660,#340,#341),#493,.T.);
#4672=ADVANCED_FACE('',(#661,#342),#494,.T.);
#4673=ADVANCED_FACE('',(#662),#495,.T.);
#4674=ADVANCED_FACE('',(#663),#4566,.F.);
#4675=ADVANCED_FACE('',(#664),#496,.T.);
#4676=ADVANCED_FACE('',(#665),#4567,.F.);
#4677=ADVANCED_FACE('',(#666),#497,.T.);
#4965=CLOSED_SHELL('',(#4633,#4634,#4635,#4636,#4637,#4638,#4639,#4640,
#4641,#4642,#4643,#4644,#4645,#4646,#4647,#4648,#4649,#4650,#4651,#4652,
#4653,#4654,#4655,#4656,#4657,#4658,#4659,#4660,#4661,#4662,#4663,#4664,
#4665,#4666,#4667,#4668,#4669,#4670,#4671,#4672,#4673,#4674,#4675,#4676,
#4677));
#5123=AXIS2_PLACEMENT_3D('',#7472,#5828,#5829);
#5124=AXIS2_PLACEMENT_3D('',#7473,#5830,#5831);
#5125=AXIS2_PLACEMENT_3D('',#7475,#5832,#5833);
#5126=AXIS2_PLACEMENT_3D('',#7478,#5835,#5836);
#5127=AXIS2_PLACEMENT_3D('',#7479,#5837,#5838);
#5128=AXIS2_PLACEMENT_3D('',#7481,#5839,#5840);
#5129=AXIS2_PLACEMENT_3D('',#7482,#5841,#5842);
#5130=AXIS2_PLACEMENT_3D('',#7484,#5843,#5844);
#5131=AXIS2_PLACEMENT_3D('',#7487,#5846,#5847);
#5132=AXIS2_PLACEMENT_3D('',#7488,#5848,#5849);
#5133=AXIS2_PLACEMENT_3D('',#7489,#5850,#5851);
#5134=AXIS2_PLACEMENT_3D('',#7491,#5852,#5853);
#5135=AXIS2_PLACEMENT_3D('',#7494,#5855,#5856);
#5136=AXIS2_PLACEMENT_3D('',#7495,#5857,#5858);
#5137=AXIS2_PLACEMENT_3D('',#7496,#5859,#5860);
#5138=AXIS2_PLACEMENT_3D('',#7498,#5861,#5862);
#5139=AXIS2_PLACEMENT_3D('',#7501,#5864,#5865);
#5140=AXIS2_PLACEMENT_3D('',#7502,#5866,#5867);
#5141=AXIS2_PLACEMENT_3D('',#7504,#5868,#5869);
#5142=AXIS2_PLACEMENT_3D('',#7505,#5870,#5871);
#5143=AXIS2_PLACEMENT_3D('',#7508,#5873,#5874);
#5144=AXIS2_PLACEMENT_3D('',#7509,#5875,#5876);
#5145=AXIS2_PLACEMENT_3D('',#7511,#5877,#5878);
#5146=AXIS2_PLACEMENT_3D('',#7514,#5880,#5881);
#5147=AXIS2_PLACEMENT_3D('',#7515,#5882,#5883);
#5148=AXIS2_PLACEMENT_3D('',#7516,#5884,#5885);
#5149=AXIS2_PLACEMENT_3D('',#7519,#5887,#5888);
#5150=AXIS2_PLACEMENT_3D('',#7520,#5889,#5890);
#5151=AXIS2_PLACEMENT_3D('',#7525,#5892,#5893);
#5152=AXIS2_PLACEMENT_3D('',#7528,#5895,#5896);
#5153=AXIS2_PLACEMENT_3D('',#7529,#5897,#5898);
#5154=AXIS2_PLACEMENT_3D('',#7543,#5906,#5907);
#5155=AXIS2_PLACEMENT_3D('',#7551,#5911,#5912);
#5156=AXIS2_PLACEMENT_3D('',#7554,#5914,#5915);
#5157=AXIS2_PLACEMENT_3D('',#7555,#5916,#5917);
#5158=AXIS2_PLACEMENT_3D('',#7558,#5919,#5920);
#5159=AXIS2_PLACEMENT_3D('',#7559,#5921,#5922);
#5160=AXIS2_PLACEMENT_3D('',#7561,#5923,#5924);
#5161=AXIS2_PLACEMENT_3D('',#7565,#5926,#5927);
#5162=AXIS2_PLACEMENT_3D('',#7569,#5930,#5931);
#5163=AXIS2_PLACEMENT_3D('',#7572,#5933,#5934);
#5164=AXIS2_PLACEMENT_3D('',#7573,#5935,#5936);
#5165=AXIS2_PLACEMENT_3D('',#7577,#5939,#5940);
#5166=AXIS2_PLACEMENT_3D('',#7580,#5942,#5943);
#5167=AXIS2_PLACEMENT_3D('',#7581,#5944,#5945);
#5168=AXIS2_PLACEMENT_3D('',#7585,#5947,#5948);
#5169=AXIS2_PLACEMENT_3D('',#7587,#5950,#5951);
#5170=AXIS2_PLACEMENT_3D('',#7590,#5952,#5953);
#5171=AXIS2_PLACEMENT_3D('',#7592,#5954,#5955);
#5172=AXIS2_PLACEMENT_3D('',#7593,#5956,#5957);
#5173=AXIS2_PLACEMENT_3D('',#7594,#5958,#5959);
#5174=AXIS2_PLACEMENT_3D('',#7596,#5960,#5961);
#5175=AXIS2_PLACEMENT_3D('',#7597,#5962,#5963);
#5176=AXIS2_PLACEMENT_3D('',#7598,#5964,#5965);
#5177=AXIS2_PLACEMENT_3D('',#7601,#5968,#5969);
#5178=AXIS2_PLACEMENT_3D('',#7604,#5970,#5971);
#5179=AXIS2_PLACEMENT_3D('',#7605,#5972,#5973);
#5180=AXIS2_PLACEMENT_3D('',#7606,#5974,#5975);
#5181=AXIS2_PLACEMENT_3D('',#7607,#5976,#5977);
#5182=AXIS2_PLACEMENT_3D('',#7609,#5978,#5979);
#5183=AXIS2_PLACEMENT_3D('',#7610,#5980,#5981);
#5184=AXIS2_PLACEMENT_3D('',#7611,#5982,#5983);
#5185=AXIS2_PLACEMENT_3D('',#7616,#5986,#5987);
#5186=AXIS2_PLACEMENT_3D('',#7617,#5988,#5989);
#5187=AXIS2_PLACEMENT_3D('',#7619,#5990,#5991);
#5188=AXIS2_PLACEMENT_3D('',#7621,#5992,#5993);
#5189=AXIS2_PLACEMENT_3D('',#7622,#5994,#5995);
#5190=AXIS2_PLACEMENT_3D('',#7623,#5996,#5997);
#5191=AXIS2_PLACEMENT_3D('',#7625,#5999,#6000);
#5192=AXIS2_PLACEMENT_3D('',#7628,#6003,#6004);
#5193=AXIS2_PLACEMENT_3D('',#7630,#6005,#6006);
#5194=AXIS2_PLACEMENT_3D('',#7631,#6007,#6008);
#5195=AXIS2_PLACEMENT_3D('',#7632,#6009,#6010);
#5196=AXIS2_PLACEMENT_3D('',#7635,#6012,#6013);
#5197=AXIS2_PLACEMENT_3D('',#7636,#6014,#6015);
#5198=AXIS2_PLACEMENT_3D('',#7638,#6017,#6018);
#5199=AXIS2_PLACEMENT_3D('',#7640,#6020,#6021);
#5200=AXIS2_PLACEMENT_3D('',#7642,#6023,#6024);
#5201=AXIS2_PLACEMENT_3D('',#7645,#6027,#6028);
#5202=AXIS2_PLACEMENT_3D('',#7648,#6031,#6032);
#5203=AXIS2_PLACEMENT_3D('',#7650,#6034,#6035);
#5204=AXIS2_PLACEMENT_3D('',#7651,#6036,#6037);
#5205=AXIS2_PLACEMENT_3D('',#7653,#6038,#6039);
#5206=AXIS2_PLACEMENT_3D('',#7654,#6040,#6041);
#5207=AXIS2_PLACEMENT_3D('',#7655,#6042,#6043);
#5208=AXIS2_PLACEMENT_3D('',#7656,#6044,#6045);
#5209=AXIS2_PLACEMENT_3D('',#7657,#6046,#6047);
#5210=AXIS2_PLACEMENT_3D('',#7659,#6048,#6049);
#5211=AXIS2_PLACEMENT_3D('',#7660,#6050,#6051);
#5212=AXIS2_PLACEMENT_3D('',#7662,#6053,#6054);
#5828=DIRECTION('axis',(0.,0.,1.));
#5829=DIRECTION('refdir',(1.,0.,0.));
#5830=DIRECTION('center_axis',(-1.,0.,0.));
#5831=DIRECTION('ref_axis',(0.,1.,0.));
#5832=DIRECTION('center_axis',(-1.,0.,0.));
#5833=DIRECTION('ref_axis',(0.,1.,0.));
#5834=DIRECTION('',(-1.,0.,0.));
#5835=DIRECTION('center_axis',(-1.,0.,0.));
#5836=DIRECTION('ref_axis',(0.,1.,0.));
#5837=DIRECTION('center_axis',(1.,0.,0.));
#5838=DIRECTION('ref_axis',(0.,1.,0.));
#5839=DIRECTION('center_axis',(1.,0.,0.));
#5840=DIRECTION('ref_axis',(0.,1.,0.));
#5841=DIRECTION('center_axis',(0.,0.,-1.));
#5842=DIRECTION('ref_axis',(1.,0.,0.));
#5843=DIRECTION('center_axis',(0.,0.,-1.));
#5844=DIRECTION('ref_axis',(1.,0.,0.));
#5845=DIRECTION('',(0.,0.,-1.));
#5846=DIRECTION('center_axis',(0.,0.,-1.));
#5847=DIRECTION('ref_axis',(1.,0.,0.));
#5848=DIRECTION('center_axis',(0.,0.,1.));
#5849=DIRECTION('ref_axis',(1.,0.,0.));
#5850=DIRECTION('center_axis',(0.,0.,-1.));
#5851=DIRECTION('ref_axis',(1.,0.,0.));
#5852=DIRECTION('center_axis',(0.,0.,-1.));
#5853=DIRECTION('ref_axis',(1.,0.,0.));
#5854=DIRECTION('',(0.,0.,-1.));
#5855=DIRECTION('center_axis',(0.,0.,-1.));
#5856=DIRECTION('ref_axis',(1.,0.,0.));
#5857=DIRECTION('center_axis',(0.,0.,1.));
#5858=DIRECTION('ref_axis',(1.,0.,0.));
#5859=DIRECTION('center_axis',(0.,1.,0.));
#5860=DIRECTION('ref_axis',(1.,0.,0.));
#5861=DIRECTION('center_axis',(0.,1.,0.));
#5862=DIRECTION('ref_axis',(1.,0.,0.));
#5863=DIRECTION('',(0.,1.,0.));
#5864=DIRECTION('center_axis',(0.,1.,0.));
#5865=DIRECTION('ref_axis',(1.,0.,0.));
#5866=DIRECTION('center_axis',(0.,-1.,0.));
#5867=DIRECTION('ref_axis',(1.,0.,0.));
#5868=DIRECTION('center_axis',(0.,-1.,0.));
#5869=DIRECTION('ref_axis',(1.,0.,0.));
#5870=DIRECTION('center_axis',(0.,1.,0.));
#5871=DIRECTION('ref_axis',(1.,0.,0.));
#5872=DIRECTION('',(0.,1.,0.));
#5873=DIRECTION('center_axis',(0.,-1.,0.));
#5874=DIRECTION('ref_axis',(1.,0.,0.));
#5875=DIRECTION('center_axis',(0.,1.,0.));
#5876=DIRECTION('ref_axis',(1.,0.,0.));
#5877=DIRECTION('center_axis',(0.,1.,0.));
#5878=DIRECTION('ref_axis',(1.,0.,0.));
#5879=DIRECTION('',(0.,1.,0.));
#5880=DIRECTION('center_axis',(0.,1.,0.));
#5881=DIRECTION('ref_axis',(1.,0.,0.));
#5882=DIRECTION('center_axis',(0.,-1.,0.));
#5883=DIRECTION('ref_axis',(1.,0.,0.));
#5884=DIRECTION('center_axis',(-1.,0.,0.));
#5885=DIRECTION('ref_axis',(0.,1.,0.));
#5886=DIRECTION('',(-1.,0.,0.));
#5887=DIRECTION('center_axis',(1.,0.,0.));
#5888=DIRECTION('ref_axis',(0.,1.,0.));
#5889=DIRECTION('center_axis',(1.,0.,0.));
#5890=DIRECTION('ref_axis',(0.,-6.12323399573677E-17,-1.));
#5891=DIRECTION('',(-1.,0.,0.));
#5892=DIRECTION('center_axis',(-1.,0.,0.));
#5893=DIRECTION('ref_axis',(0.,-1.,0.));
#5894=DIRECTION('',(1.,0.,0.));
#5895=DIRECTION('center_axis',(1.,0.,0.));
#5896=DIRECTION('ref_axis',(0.,-1.,0.));
#5897=DIRECTION('center_axis',(-1.,0.,0.));
#5898=DIRECTION('ref_axis',(0.,-1.,0.));
#5899=DIRECTION('',(0.,0.,1.));
#5900=DIRECTION('',(0.,-1.,0.));
#5901=DIRECTION('',(0.,0.,1.));
#5902=DIRECTION('',(0.,1.,0.));
#5903=DIRECTION('',(0.,0.,-1.));
#5904=DIRECTION('',(0.,-1.,0.));
#5905=DIRECTION('',(0.,0.,-1.));
#5906=DIRECTION('center_axis',(0.,1.,0.));
#5907=DIRECTION('ref_axis',(1.,0.,0.));
#5908=DIRECTION('',(0.,0.,-1.));
#5909=DIRECTION('',(-1.,0.,0.));
#5910=DIRECTION('',(0.,0.,-1.));
#5911=DIRECTION('center_axis',(0.,1.,0.));
#5912=DIRECTION('ref_axis',(0.70710678118654,0.,0.707106781186555));
#5913=DIRECTION('',(1.,0.,0.));
#5914=DIRECTION('center_axis',(0.,1.,0.));
#5915=DIRECTION('ref_axis',(-0.70710678118654,0.,0.707106781186555));
#5916=DIRECTION('center_axis',(1.,0.,0.));
#5917=DIRECTION('ref_axis',(0.,1.,0.));
#5918=DIRECTION('',(0.,0.,1.));
#5919=DIRECTION('center_axis',(-1.,0.,0.));
#5920=DIRECTION('ref_axis',(0.,1.,0.));
#5921=DIRECTION('center_axis',(0.,-1.,0.));
#5922=DIRECTION('ref_axis',(-1.,0.,0.));
#5923=DIRECTION('center_axis',(0.,-1.,0.));
#5924=DIRECTION('ref_axis',(-0.70710678118654,0.,0.707106781186555));
#5925=DIRECTION('',(-1.,0.,0.));
#5926=DIRECTION('center_axis',(0.,-1.,0.));
#5927=DIRECTION('ref_axis',(0.70710678118654,0.,0.707106781186555));
#5928=DIRECTION('',(0.,0.,1.));
#5929=DIRECTION('',(1.,0.,0.));
#5930=DIRECTION('center_axis',(0.,-1.,0.));
#5931=DIRECTION('ref_axis',(-0.70710678118654,0.,0.707106781186555));
#5932=DIRECTION('',(0.,1.,0.));
#5933=DIRECTION('center_axis',(0.,1.,0.));
#5934=DIRECTION('ref_axis',(0.,0.,1.));
#5935=DIRECTION('center_axis',(0.,0.,1.));
#5936=DIRECTION('ref_axis',(1.,0.,0.));
#5937=DIRECTION('',(0.,-1.,0.));
#5938=DIRECTION('',(1.,0.,0.));
#5939=DIRECTION('center_axis',(0.,1.,0.));
#5940=DIRECTION('ref_axis',(0.70710678118654,0.,0.707106781186555));
#5941=DIRECTION('',(0.,1.,0.));
#5942=DIRECTION('center_axis',(0.,1.,0.));
#5943=DIRECTION('ref_axis',(1.,0.,0.));
#5944=DIRECTION('center_axis',(0.,1.,0.));
#5945=DIRECTION('ref_axis',(0.70710678118654,0.,0.707106781186555));
#5946=DIRECTION('',(0.,-1.,0.));
#5947=DIRECTION('center_axis',(0.,-1.,0.));
#5948=DIRECTION('ref_axis',(0.,0.,1.));
#5949=DIRECTION('',(0.,1.,0.));
#5950=DIRECTION('center_axis',(-0.40824829046386,-0.816496580927727,0.408248290463864));
#5951=DIRECTION('ref_axis',(0.577350269189625,-0.577350269189625,-0.577350269189628));
#5952=DIRECTION('center_axis',(0.,-1.,0.));
#5953=DIRECTION('ref_axis',(1.,0.,0.));
#5954=DIRECTION('center_axis',(0.,0.,-1.));
#5955=DIRECTION('ref_axis',(0.,-1.,0.));
#5956=DIRECTION('center_axis',(1.,0.,0.));
#5957=DIRECTION('ref_axis',(0.,0.,-1.));
#5958=DIRECTION('center_axis',(-0.40824829046386,-0.816496580927727,-0.408248290463864));
#5959=DIRECTION('ref_axis',(0.577350269189625,-0.577350269189625,0.577350269189628));
#5960=DIRECTION('center_axis',(1.,0.,0.));
#5961=DIRECTION('ref_axis',(0.,-1.,0.));
#5962=DIRECTION('center_axis',(0.,0.,1.));
#5963=DIRECTION('ref_axis',(1.,0.,0.));
#5964=DIRECTION('center_axis',(0.,0.,1.));
#5965=DIRECTION('ref_axis',(0.707106781186541,-0.707106781186554,0.));
#5966=DIRECTION('',(0.,0.,-1.));
#5967=DIRECTION('',(0.,0.,1.));
#5968=DIRECTION('center_axis',(0.40824829046386,-0.816496580927727,0.408248290463864));
#5969=DIRECTION('ref_axis',(-0.577350269189625,-0.577350269189625,-0.577350269189628));
#5970=DIRECTION('center_axis',(-1.,0.,0.));
#5971=DIRECTION('ref_axis',(0.,-1.,0.));
#5972=DIRECTION('center_axis',(0.,0.,-1.));
#5973=DIRECTION('ref_axis',(-1.,0.,0.));
#5974=DIRECTION('center_axis',(0.,-1.,0.));
#5975=DIRECTION('ref_axis',(0.,0.,-1.));
#5976=DIRECTION('center_axis',(0.408248290463862,0.408248290463855,-0.816496580927731));
#5977=DIRECTION('ref_axis',(0.577350269189628,0.577350269189628,0.577350269189621));
#5978=DIRECTION('center_axis',(0.,0.,1.));
#5979=DIRECTION('ref_axis',(0.,1.,0.));
#5980=DIRECTION('center_axis',(1.,1.77635683940026E-14,0.));
#5981=DIRECTION('ref_axis',(0.,0.,1.));
#5982=DIRECTION('center_axis',(0.,0.,1.));
#5983=DIRECTION('ref_axis',(0.707106781186554,0.707106781186541,0.));
#5984=DIRECTION('',(0.,0.,1.));
#5985=DIRECTION('',(0.,0.,-1.));
#5986=DIRECTION('center_axis',(0.,0.707106781186549,0.707106781186546));
#5987=DIRECTION('ref_axis',(0.,0.707106781186546,-0.707106781186549));
#5988=DIRECTION('center_axis',(0.40824829046386,-0.816496580927727,-0.408248290463864));
#5989=DIRECTION('ref_axis',(-0.577350269189625,-0.577350269189625,0.577350269189628));
#5990=DIRECTION('center_axis',(0.,-1.,0.));
#5991=DIRECTION('ref_axis',(-1.,0.,0.));
#5992=DIRECTION('center_axis',(0.,0.,1.));
#5993=DIRECTION('ref_axis',(0.,-1.,0.));
#5994=DIRECTION('center_axis',(-1.,0.,0.));
#5995=DIRECTION('ref_axis',(0.,0.,1.));
#5996=DIRECTION('center_axis',(0.,0.,-1.));
#5997=DIRECTION('ref_axis',(-0.707106781186541,-0.707106781186554,0.));
#5998=DIRECTION('',(0.,0.,1.));
#5999=DIRECTION('center_axis',(1.,0.,0.));
#6000=DIRECTION('ref_axis',(0.,-0.707106781186546,0.707106781186549));
#6001=DIRECTION('',(-1.,0.,0.));
#6002=DIRECTION('',(1.,0.,0.));
#6003=DIRECTION('center_axis',(-0.40824829046386,-0.816496580927727,0.408248290463864));
#6004=DIRECTION('ref_axis',(-0.577350269189625,0.577350269189625,0.577350269189628));
#6005=DIRECTION('center_axis',(-1.,0.,0.));
#6006=DIRECTION('ref_axis',(0.,1.,0.));
#6007=DIRECTION('center_axis',(0.,0.,1.));
#6008=DIRECTION('ref_axis',(-1.,0.,0.));
#6009=DIRECTION('center_axis',(0.,0.,1.));
#6010=DIRECTION('ref_axis',(-0.707106781186541,0.707106781186554,0.));
#6011=DIRECTION('',(0.,0.,-1.));
#6012=DIRECTION('center_axis',(0.,0.707106781186549,0.707106781186546));
#6013=DIRECTION('ref_axis',(0.,0.707106781186546,-0.707106781186549));
#6014=DIRECTION('center_axis',(0.,-1.,0.));
#6015=DIRECTION('ref_axis',(-0.70710678118654,0.,0.707106781186555));
#6016=DIRECTION('',(0.,1.,0.));
#6017=DIRECTION('center_axis',(-1.,0.,0.));
#6018=DIRECTION('ref_axis',(0.,0.707106781186546,0.707106781186549));
#6019=DIRECTION('',(-1.,0.,0.));
#6020=DIRECTION('center_axis',(0.,1.,0.));
#6021=DIRECTION('ref_axis',(-0.70710678118654,0.,-0.707106781186555));
#6022=DIRECTION('',(0.,-1.,0.));
#6023=DIRECTION('center_axis',(-1.,0.,0.));
#6024=DIRECTION('ref_axis',(0.,-0.707106781186546,-0.707106781186549));
#6025=DIRECTION('',(1.,0.,0.));
#6026=DIRECTION('',(-1.,0.,0.));
#6027=DIRECTION('center_axis',(0.,-1.,0.));
#6028=DIRECTION('ref_axis',(0.70710678118654,0.,-0.707106781186555));
#6029=DIRECTION('',(0.,-1.,0.));
#6030=DIRECTION('',(0.,1.,0.));
#6031=DIRECTION('center_axis',(0.,0.,-1.));
#6032=DIRECTION('ref_axis',(-1.,0.,0.));
#6033=DIRECTION('',(1.,0.,0.));
#6034=DIRECTION('center_axis',(1.,0.,0.));
#6035=DIRECTION('ref_axis',(0.,1.,0.));
#6036=DIRECTION('center_axis',(-1.,0.,0.));
#6037=DIRECTION('ref_axis',(0.,1.,0.));
#6038=DIRECTION('center_axis',(-1.,0.,0.));
#6039=DIRECTION('ref_axis',(0.,1.,0.));
#6040=DIRECTION('center_axis',(0.,-1.,0.));
#6041=DIRECTION('ref_axis',(1.,0.,0.));
#6042=DIRECTION('center_axis',(0.,0.,1.));
#6043=DIRECTION('ref_axis',(1.,0.,0.));
#6044=DIRECTION('center_axis',(1.,0.,0.));
#6045=DIRECTION('ref_axis',(0.,-1.83697019872103E-16,-1.));
#6046=DIRECTION('center_axis',(1.,0.,0.));
#6047=DIRECTION('ref_axis',(0.,1.,0.));
#6048=DIRECTION('center_axis',(-1.,0.,0.));
#6049=DIRECTION('ref_axis',(0.,1.,0.));
#6050=DIRECTION('center_axis',(1.,0.,0.));
#6051=DIRECTION('ref_axis',(0.,1.,0.));
#6052=DIRECTION('',(1.,0.,0.));
#6053=DIRECTION('center_axis',(0.,1.,0.));
#6054=DIRECTION('ref_axis',(-1.,0.,0.));
#7472=CARTESIAN_POINT('',(0.,0.,0.));
#7473=CARTESIAN_POINT('Origin',(140.,37.8343839603864,-8.00000000000001));
#7474=CARTESIAN_POINT('',(-130.,31.8343839603864,-8.00000000000001));
#7475=CARTESIAN_POINT('Origin',(-130.,37.8343839603864,-8.00000000000001));
#7476=CARTESIAN_POINT('',(-145.,31.8343839603864,-8.00000000000001));
#7477=CARTESIAN_POINT('',(140.,31.8343839603864,-8.00000000000001));
#7478=CARTESIAN_POINT('Origin',(-145.,37.8343839603864,-8.00000000000001));
#7479=CARTESIAN_POINT('Origin',(-145.,37.8343839603864,-8.00000000000001));
#7480=CARTESIAN_POINT('',(-145.,32.8343839603866,-8.00000000000001));
#7481=CARTESIAN_POINT('Origin',(-145.,37.8343839603864,-8.00000000000001));
#7482=CARTESIAN_POINT('Origin',(-140.,-23.6740181268338,20.));
#7483=CARTESIAN_POINT('',(-144.,-23.6740181268338,20.));
#7484=CARTESIAN_POINT('Origin',(-140.,-23.6740181268338,20.));
#7485=CARTESIAN_POINT('',(-144.,-23.6740181268338,0.));
#7486=CARTESIAN_POINT('',(-144.,-23.6740181268338,20.));
#7487=CARTESIAN_POINT('Origin',(-140.,-23.6740181268338,0.));
#7488=CARTESIAN_POINT('Origin',(-140.,-23.6740181268338,0.));
#7489=CARTESIAN_POINT('Origin',(-140.,23.6740181268338,20.));
#7490=CARTESIAN_POINT('',(-144.,23.6740181268338,20.));
#7491=CARTESIAN_POINT('Origin',(-140.,23.6740181268338,20.));
#7492=CARTESIAN_POINT('',(-144.,23.6740181268338,0.));
#7493=CARTESIAN_POINT('',(-144.,23.6740181268338,20.));
#7494=CARTESIAN_POINT('Origin',(-140.,23.6740181268338,0.));
#7495=CARTESIAN_POINT('Origin',(-140.,23.6740181268338,0.));
#7496=CARTESIAN_POINT('Origin',(-140.,-50.,8.77546295170414));
#7497=CARTESIAN_POINT('',(-145.,-50.,8.77546295170414));
#7498=CARTESIAN_POINT('Origin',(-140.,-50.,8.77546295170414));
#7499=CARTESIAN_POINT('',(-145.,-42.,8.77546295170414));
#7500=CARTESIAN_POINT('',(-145.,-50.,8.77546295170414));
#7501=CARTESIAN_POINT('Origin',(-140.,-42.,8.77546295170414));
#7502=CARTESIAN_POINT('Origin',(-140.,-42.,8.77546295170414));
#7503=CARTESIAN_POINT('',(-143.,-42.,8.77546295170414));
#7504=CARTESIAN_POINT('Origin',(-140.,-42.,8.77546295170414));
#7505=CARTESIAN_POINT('Origin',(-140.,-50.,8.77546295170414));
#7506=CARTESIAN_POINT('',(-143.,-38.3343839603864,8.77546295170414));
#7507=CARTESIAN_POINT('',(-143.,-50.,8.77546295170414));
#7508=CARTESIAN_POINT('Origin',(-140.,-38.3343839603864,8.77546295170414));
#7509=CARTESIAN_POINT('Origin',(-140.,-50.,8.77546295170414));
#7510=CARTESIAN_POINT('',(-143.,-37.3343839603864,8.77546295170414));
#7511=CARTESIAN_POINT('Origin',(-140.,-37.3343839603864,8.77546295170414));
#7512=CARTESIAN_POINT('',(-143.,-30.,8.77546295170414));
#7513=CARTESIAN_POINT('',(-143.,-50.,8.77546295170414));
#7514=CARTESIAN_POINT('Origin',(-140.,-30.,8.77546295170414));
#7515=CARTESIAN_POINT('Origin',(-140.,-30.,8.77546295170414));
#7516=CARTESIAN_POINT('Origin',(-150.,37.8343839603864,-8.00000000000001));
#7517=CARTESIAN_POINT('',(-150.,32.8343839603866,-8.00000000000001));
#7518=CARTESIAN_POINT('',(-150.,32.8343839603866,-8.00000000000001));
#7519=CARTESIAN_POINT('Origin',(-150.,37.8343839603864,-8.00000000000001));
#7520=CARTESIAN_POINT('Origin',(-150.,-37.8343839603864,-8.00000000000001));
#7521=CARTESIAN_POINT('',(-140.,-38.3343839603864,-3.02506281446715));
#7522=CARTESIAN_POINT('',(-150.,-38.3343839603864,-3.02506281446715));
#7523=CARTESIAN_POINT('',(-150.,-38.3343839603864,-3.02506281446715));
#7524=CARTESIAN_POINT('',(-140.,-37.3343839603864,-3.02506281446715));
#7525=CARTESIAN_POINT('Origin',(-140.,-37.8343839603864,-8.00000000000001));
#7526=CARTESIAN_POINT('',(-150.,-37.3343839603864,-3.02506281446715));
#7527=CARTESIAN_POINT('',(-150.,-37.3343839603864,-3.02506281446715));
#7528=CARTESIAN_POINT('Origin',(-150.,-37.8343839603864,-8.00000000000001));
#7529=CARTESIAN_POINT('Origin',(-150.,50.,0.));
#7530=CARTESIAN_POINT('',(-150.,-37.3343839603864,19.));
#7531=CARTESIAN_POINT('',(-150.,-37.3343839603864,10.));
#7532=CARTESIAN_POINT('',(-150.,49.,19.));
#7533=CARTESIAN_POINT('',(-150.,25.,19.));
#7534=CARTESIAN_POINT('',(-150.,49.,-19.));
#7535=CARTESIAN_POINT('',(-150.,49.,0.));
#7536=CARTESIAN_POINT('',(-150.,-49.,-19.));
#7537=CARTESIAN_POINT('',(-150.,25.,-19.));
#7538=CARTESIAN_POINT('',(-150.,-49.,19.));
#7539=CARTESIAN_POINT('',(-150.,-49.,0.));
#7540=CARTESIAN_POINT('',(-150.,-38.3343839603864,19.));
#7541=CARTESIAN_POINT('',(-150.,25.,19.));
#7542=CARTESIAN_POINT('',(-150.,-38.3343839603864,10.));
#7543=CARTESIAN_POINT('Origin',(-155.071229108474,-37.3343839603864,20.));
#7544=CARTESIAN_POINT('',(-140.,-37.3343839603864,-2.02086962844929));
#7545=CARTESIAN_POINT('',(-140.,-37.3343839603864,6.));
#7546=CARTESIAN_POINT('',(-130.,-37.3343839603864,-2.02086962844929));
#7547=CARTESIAN_POINT('',(0.,-37.3343839603864,-2.02086962844929));
#7548=CARTESIAN_POINT('',(-130.,-37.3343839603864,19.));
#7549=CARTESIAN_POINT('',(-130.,-37.3343839603864,10.));
#7550=CARTESIAN_POINT('',(-131.,-37.3343839603864,20.));
#7551=CARTESIAN_POINT('Origin',(-131.,-37.3343839603864,19.));
#7552=CARTESIAN_POINT('',(-149.,-37.3343839603864,20.));
#7553=CARTESIAN_POINT('',(-147.535614554237,-37.3343839603864,20.));
#7554=CARTESIAN_POINT('Origin',(-149.,-37.3343839603864,19.));
#7555=CARTESIAN_POINT('Origin',(-140.,-37.8343839603864,-7.99999999999999));
#7556=CARTESIAN_POINT('',(-140.,-38.3343839603864,-2.02086962844929));
#7557=CARTESIAN_POINT('',(-140.,-38.3343839603864,6.));
#7558=CARTESIAN_POINT('Origin',(-140.,-37.8343839603864,-7.99999999999999));
#7559=CARTESIAN_POINT('Origin',(-124.928770891526,-38.3343839603864,20.));
#7560=CARTESIAN_POINT('',(-149.,-38.3343839603864,20.));
#7561=CARTESIAN_POINT('Origin',(-149.,-38.3343839603864,19.));
#7562=CARTESIAN_POINT('',(-131.,-38.3343839603864,20.));
#7563=CARTESIAN_POINT('',(-132.464385445763,-38.3343839603864,20.));
#7564=CARTESIAN_POINT('',(-130.,-38.3343839603864,19.));
#7565=CARTESIAN_POINT('Origin',(-131.,-38.3343839603864,19.));
#7566=CARTESIAN_POINT('',(-130.,-38.3343839603864,-2.02086962844929));
#7567=CARTESIAN_POINT('',(-130.,-38.3343839603864,10.));
#7568=CARTESIAN_POINT('',(0.,-38.3343839603864,-2.02086962844929));
#7569=CARTESIAN_POINT('Origin',(-149.,25.,19.));
#7570=CARTESIAN_POINT('',(-149.,49.,20.));
#7571=CARTESIAN_POINT('',(-149.,25.,20.));
#7572=CARTESIAN_POINT('Origin',(-149.,49.,19.));
#7573=CARTESIAN_POINT('Origin',(-140.,8.88178419700125E-15,20.));
#7574=CARTESIAN_POINT('',(-131.,49.,20.));
#7575=CARTESIAN_POINT('',(-131.,-25.,20.));
#7576=CARTESIAN_POINT('',(-135.,49.,20.));
#7577=CARTESIAN_POINT('Origin',(-131.,-25.,19.));
#7578=CARTESIAN_POINT('',(-130.,49.,19.));
#7579=CARTESIAN_POINT('',(-130.,-25.,19.));
#7580=CARTESIAN_POINT('Origin',(-131.,49.,19.));
#7581=CARTESIAN_POINT('Origin',(-131.,-25.,19.));
#7582=CARTESIAN_POINT('',(-131.,-49.,20.));
#7583=CARTESIAN_POINT('',(-131.,-25.,20.));
#7584=CARTESIAN_POINT('',(-130.,-49.,19.));
#7585=CARTESIAN_POINT('Origin',(-131.,-49.,19.));
#7586=CARTESIAN_POINT('',(-130.,-25.,19.));
#7587=CARTESIAN_POINT('Origin',(-131.,-49.,-19.));
#7588=CARTESIAN_POINT('',(-130.,-49.,-19.));
#7589=CARTESIAN_POINT('',(-131.,-49.,-20.));
#7590=CARTESIAN_POINT('Origin',(-131.,-49.,-19.));
#7591=CARTESIAN_POINT('',(-131.,-50.,-19.));
#7592=CARTESIAN_POINT('Origin',(-131.,-49.,-19.));
#7593=CARTESIAN_POINT('Origin',(-131.,-49.,-19.));
#7594=CARTESIAN_POINT('Origin',(-131.,-49.,19.));
#7595=CARTESIAN_POINT('',(-131.,-50.,19.));
#7596=CARTESIAN_POINT('Origin',(-131.,-49.,19.));
#7597=CARTESIAN_POINT('Origin',(-131.,-49.,19.));
#7598=CARTESIAN_POINT('Origin',(-131.,-49.,0.));
#7599=CARTESIAN_POINT('',(-131.,-50.,0.));
#7600=CARTESIAN_POINT('',(-130.,-49.,0.));
#7601=CARTESIAN_POINT('Origin',(-149.,-49.,-19.));
#7602=CARTESIAN_POINT('',(-149.,-50.,-19.));
#7603=CARTESIAN_POINT('',(-149.,-49.,-20.));
#7604=CARTESIAN_POINT('Origin',(-149.,-49.,-19.));
#7605=CARTESIAN_POINT('Origin',(-149.,-49.,-19.));
#7606=CARTESIAN_POINT('Origin',(-149.,-49.,-19.));
#7607=CARTESIAN_POINT('Origin',(-131.,49.,19.));
#7608=CARTESIAN_POINT('',(-131.,50.,19.));
#7609=CARTESIAN_POINT('Origin',(-131.,49.,19.));
#7610=CARTESIAN_POINT('Origin',(-131.,49.,19.));
#7611=CARTESIAN_POINT('Origin',(-131.,49.,0.));
#7612=CARTESIAN_POINT('',(-131.,50.,-20.));
#7613=CARTESIAN_POINT('',(-131.,50.,0.));
#7614=CARTESIAN_POINT('',(-130.,49.,-19.));
#7615=CARTESIAN_POINT('',(-130.,49.,0.));
#7616=CARTESIAN_POINT('Origin',(-131.,49.,-19.));
#7617=CARTESIAN_POINT('Origin',(-149.,-49.,19.));
#7618=CARTESIAN_POINT('',(-149.,-49.,20.));
#7619=CARTESIAN_POINT('Origin',(-149.,-49.,19.));
#7620=CARTESIAN_POINT('',(-149.,-50.,19.));
#7621=CARTESIAN_POINT('Origin',(-149.,-49.,19.));
#7622=CARTESIAN_POINT('Origin',(-149.,-49.,19.));
#7623=CARTESIAN_POINT('Origin',(-149.,-49.,0.));
#7624=CARTESIAN_POINT('',(-149.,-50.,0.));
#7625=CARTESIAN_POINT('Origin',(-145.,-49.,19.));
#7626=CARTESIAN_POINT('',(-145.,-49.,20.));
#7627=CARTESIAN_POINT('',(-145.,-50.,19.));
#7628=CARTESIAN_POINT('Origin',(-149.,49.,19.));
#7629=CARTESIAN_POINT('',(-149.,50.,19.));
#7630=CARTESIAN_POINT('Origin',(-149.,49.,19.));
#7631=CARTESIAN_POINT('Origin',(-149.,49.,19.));
#7632=CARTESIAN_POINT('Origin',(-149.,49.,0.));
#7633=CARTESIAN_POINT('',(-149.,50.,-20.));
#7634=CARTESIAN_POINT('',(-149.,50.,0.));
#7635=CARTESIAN_POINT('Origin',(-149.,49.,-19.));
#7636=CARTESIAN_POINT('Origin',(-149.,25.,19.));
#7637=CARTESIAN_POINT('',(-149.,25.,20.));
#7638=CARTESIAN_POINT('Origin',(-135.,49.,19.));
#7639=CARTESIAN_POINT('',(-135.,50.,19.));
#7640=CARTESIAN_POINT('Origin',(-149.,25.,-19.));
#7641=CARTESIAN_POINT('',(-149.,25.,-20.));
#7642=CARTESIAN_POINT('Origin',(-145.,-49.,-19.));
#7643=CARTESIAN_POINT('',(-145.,-49.,-20.));
#7644=CARTESIAN_POINT('',(-145.,-50.,-19.));
#7645=CARTESIAN_POINT('Origin',(-131.,-25.,-19.));
#7646=CARTESIAN_POINT('',(-130.,-25.,-19.));
#7647=CARTESIAN_POINT('',(-131.,-25.,-20.));
#7648=CARTESIAN_POINT('Origin',(-140.,8.88178419700125E-15,-20.));
#7649=CARTESIAN_POINT('',(-150.,50.,-20.));
#7650=CARTESIAN_POINT('Origin',(-130.,-50.,0.));
#7651=CARTESIAN_POINT('Origin',(-130.,-37.8343839603864,-7.99999999999999));
#7652=CARTESIAN_POINT('',(-130.,-7.50000000000001,1.14489504879301E-14));
#7653=CARTESIAN_POINT('Origin',(-130.,1.91963385766348E-15,1.05304653885696E-14));
#7654=CARTESIAN_POINT('Origin',(-150.,-50.,0.));
#7655=CARTESIAN_POINT('Origin',(-140.,8.88178419700125E-15,20.));
#7656=CARTESIAN_POINT('Origin',(0.,-37.8343839603864,-7.99999999999999));
#7657=CARTESIAN_POINT('Origin',(-140.,2.22044604925031E-15,9.99200722162641E-15));
#7658=CARTESIAN_POINT('',(-140.,-7.50000000000001,9.6119802892091E-15));
#7659=CARTESIAN_POINT('Origin',(-140.,1.91963385766348E-15,1.05304653885696E-14));
#7660=CARTESIAN_POINT('Origin',(0.,1.91963385766348E-15,1.05304653885696E-14));
#7661=CARTESIAN_POINT('',(0.,-7.50000000000001,9.61198028920908E-15));
#7662=CARTESIAN_POINT('Origin',(-130.,50.,0.));
#9476=UNCERTAINTY_MEASURE_WITH_UNIT(LENGTH_MEASURE(0.01),#9497,
'DISTANCE_ACCURACY_VALUE',
'Maximum model space distance between geometric entities at asserted c
onnectivities');
#9485=UNCERTAINTY_MEASURE_WITH_UNIT(LENGTH_MEASURE(0.01),#9497,
'DISTANCE_ACCURACY_VALUE',
'Maximum model space distance between geometric entities at asserted c
onnectivities');
#9487=(
GEOMETRIC_REPRESENTATION_CONTEXT(3)
GLOBAL_UNCERTAINTY_ASSIGNED_CONTEXT((#9476))
GLOBAL_UNIT_ASSIGNED_CONTEXT((#9497,#9499,#9500))
REPRESENTATION_CONTEXT('','3D')
);
#9496=(
GEOMETRIC_REPRESENTATION_CONTEXT(3)
GLOBAL_UNCERTAINTY_ASSIGNED_CONTEXT((#9485))
GLOBAL_UNIT_ASSIGNED_CONTEXT((#9497,#9499,#9500))
REPRESENTATION_CONTEXT('','3D')
);
#9497=(
LENGTH_UNIT()
NAMED_UNIT(*)
SI_UNIT(.MILLI.,.METRE.)
);
#9499=(
NAMED_UNIT(*)
PLANE_ANGLE_UNIT()
SI_UNIT($,.RADIAN.)
);
#9500=(
NAMED_UNIT(*)
SI_UNIT($,.STERADIAN.)
SOLID_ANGLE_UNIT()
);
#9502=SHAPE_DEFINITION_REPRESENTATION(#9512,#9539);
#9512=PRODUCT_DEFINITION_SHAPE('',$,#9550);
#9539=SHAPE_REPRESENTATION('',(#5123),#9487);
#9548=PRODUCT_DEFINITION_CONTEXT('part definition',#9580,'design');
#9550=PRODUCT_DEFINITION('End_plates_02','End_plates_02',#9560,#9548);
#9560=PRODUCT_DEFINITION_FORMATION('',$,#9583);
#9580=APPLICATION_CONTEXT(
'Core Data for Automotive Mechanical Design Process');
#9581=PRODUCT_CONTEXT('part definition',#9580,'mechanical');
#9583=PRODUCT('End_plates_02','End_plates_02',$,(#9581));
#9593=PRESENTATION_STYLE_ASSIGNMENT((#9596));
#9596=SURFACE_STYLE_USAGE(.BOTH.,#9599);
#9599=SURFACE_SIDE_STYLE('',(#9602));
#9602=SURFACE_STYLE_FILL_AREA(#9605);
#9605=FILL_AREA_STYLE('Opaque(245,245,246)',(#9608));
#9608=FILL_AREA_STYLE_COLOUR('Opaque(245,245,246)',#9611);
#9611=COLOUR_RGB('Opaque(245,245,246)', 0.66274510, 0.83137255, 0.94901961);
ENDSEC;
END-ISO-10303-21;
